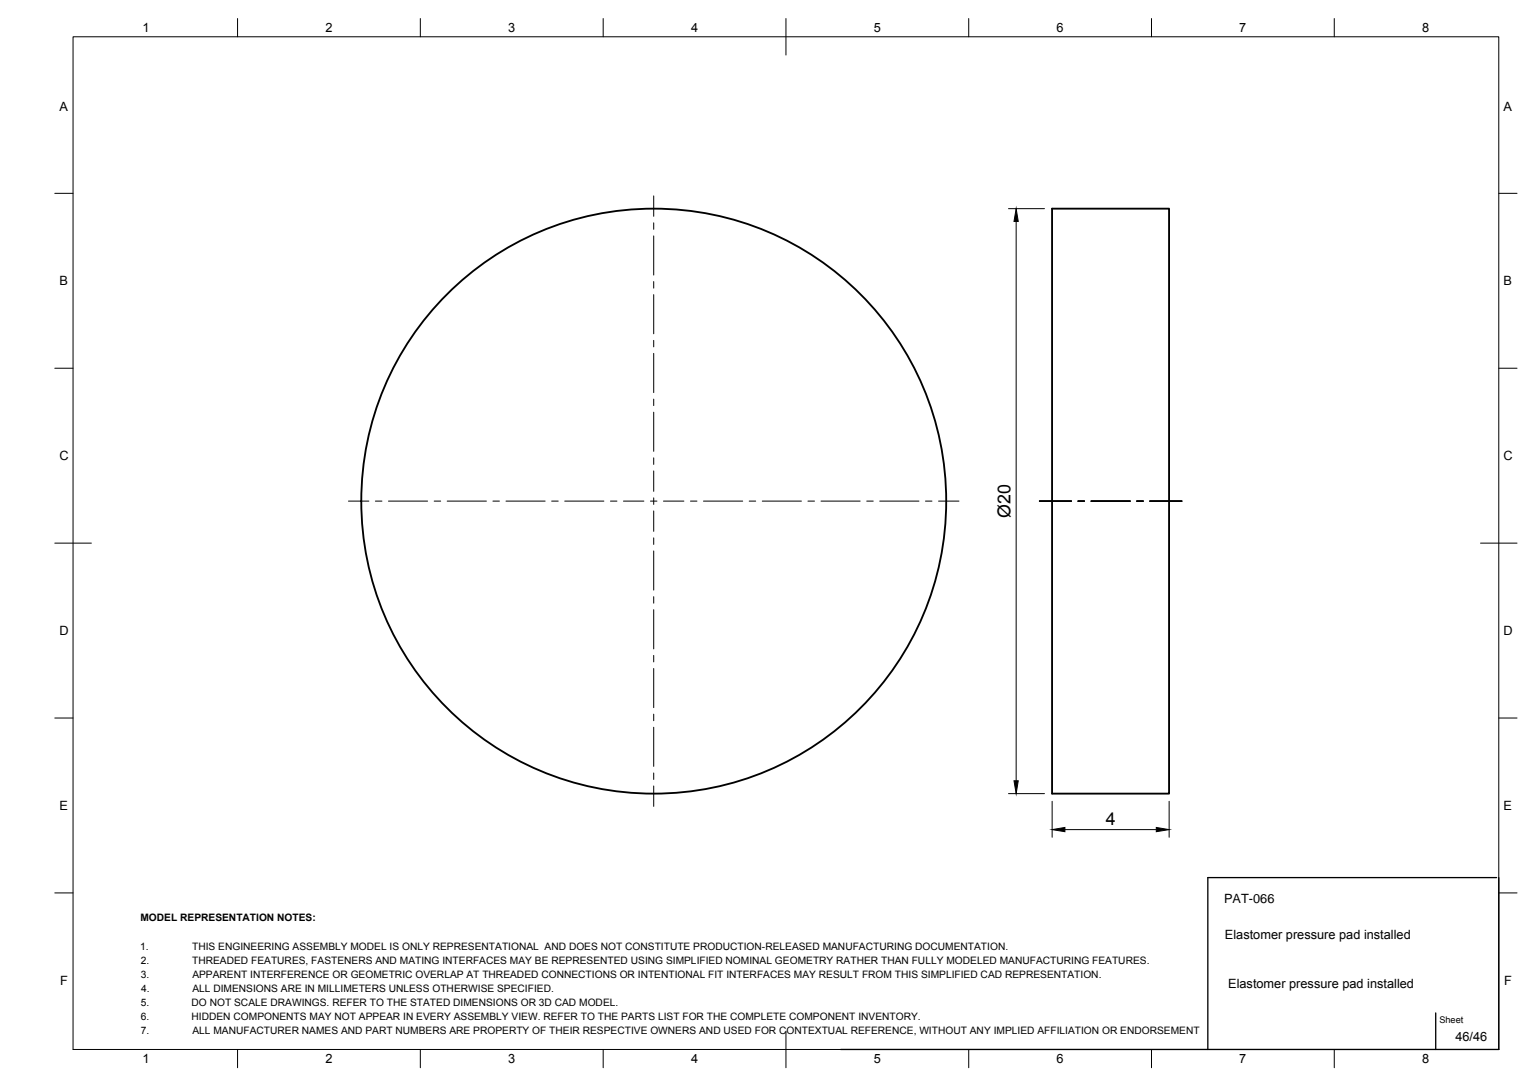
ISO-10303-21;
HEADER;
/* Generated by software containing ST-Developer
 * from STEP Tools, Inc. (www.steptools.com) 
 */

FILE_DESCRIPTION(
/* description */ ('Lever-operated bar clamp (toggle)'),
/* implementation_level */ '2;1');

FILE_NAME(
/* name */ 'Elastomer pressure pad installed.step',
/* time_stamp */ '2026-10-28T03:25:02-07:00',
/* author */ (''),
/* organization */ (''),
/* preprocessor_version */ 'ST-DEVELOPER v20.2',
/* originating_system */ 'Autodesk Translation Framework v15.17.0.0',
/* authorisation */ '');

FILE_SCHEMA (('AUTOMOTIVE_DESIGN { 1 0 10303 214 3 1 1 }'));
ENDSEC;

DATA;
#10=MECHANICAL_DESIGN_GEOMETRIC_PRESENTATION_REPRESENTATION('',(#455),#12413);
#370=SHAPE_REPRESENTATION_RELATIONSHIP('SRR','None',#12614,#408);
#408=ADVANCED_BREP_SHAPE_REPRESENTATION('',(#498),#12411);
#455=STYLED_ITEM('',(#12883),#498);
#498=MANIFOLD_SOLID_BREP('Body1',#6618);
#877=PLANE('',#7867);
#878=PLANE('',#7868);
#1279=FACE_OUTER_BOUND('',#1835,.T.);
#1280=FACE_OUTER_BOUND('',#1836,.T.);
#1281=FACE_OUTER_BOUND('',#1837,.T.);
#1835=EDGE_LOOP('',(#5977,#5978,#5979,#5980));
#1836=EDGE_LOOP('',(#5981));
#1837=EDGE_LOOP('',(#5982));
#2270=LINE('',#12256,#2711);
#2711=VECTOR('',#9967,1.);
#3068=CIRCLE('',#7865,1.);
#3069=CIRCLE('',#7866,1.);
#3597=VERTEX_POINT('',#12253);
#3598=VERTEX_POINT('',#12255);
#4393=EDGE_CURVE('',#3597,#3597,#3068,.T.);
#4394=EDGE_CURVE('',#3597,#3598,#2270,.T.);
#4395=EDGE_CURVE('',#3598,#3598,#3069,.T.);
#5977=ORIENTED_EDGE('',*,*,#4393,.F.);
#5978=ORIENTED_EDGE('',*,*,#4394,.T.);
#5979=ORIENTED_EDGE('',*,*,#4395,.T.);
#5980=ORIENTED_EDGE('',*,*,#4394,.F.);
#5981=ORIENTED_EDGE('',*,*,#4393,.T.);
#5982=ORIENTED_EDGE('',*,*,#4395,.F.);
#6161=CYLINDRICAL_SURFACE('',#7864,1.);
#6554=ADVANCED_FACE('',(#1279),#6161,.T.);
#6555=ADVANCED_FACE('',(#1280),#877,.T.);
#6556=ADVANCED_FACE('',(#1281),#878,.F.);
#6618=CLOSED_SHELL('',(#6554,#6555,#6556));
#7863=AXIS2_PLACEMENT_3D('',#12251,#9961,#9962);
#7864=AXIS2_PLACEMENT_3D('',#12252,#9963,#9964);
#7865=AXIS2_PLACEMENT_3D('',#12254,#9965,#9966);
#7866=AXIS2_PLACEMENT_3D('',#12257,#9968,#9969);
#7867=AXIS2_PLACEMENT_3D('',#12258,#9970,#9971);
#7868=AXIS2_PLACEMENT_3D('',#12259,#9972,#9973);
#9961=DIRECTION('axis',(0.,0.,1.));
#9962=DIRECTION('refdir',(1.,0.,0.));
#9963=DIRECTION('center_axis',(0.,0.,1.));
#9964=DIRECTION('ref_axis',(1.,0.,0.));
#9965=DIRECTION('center_axis',(0.,0.,1.));
#9966=DIRECTION('ref_axis',(1.,0.,0.));
#9967=DIRECTION('',(0.,0.,-1.));
#9968=DIRECTION('center_axis',(0.,0.,1.));
#9969=DIRECTION('ref_axis',(1.,0.,0.));
#9970=DIRECTION('center_axis',(0.,0.,1.));
#9971=DIRECTION('ref_axis',(1.,0.,0.));
#9972=DIRECTION('center_axis',(0.,0.,1.));
#9973=DIRECTION('ref_axis',(1.,0.,0.));
#12251=CARTESIAN_POINT('',(0.,0.,0.));
#12252=CARTESIAN_POINT('Origin',(0.,0.,3.));
#12253=CARTESIAN_POINT('',(-1.,-1.22464679914735E-16,3.4));
#12254=CARTESIAN_POINT('Origin',(0.,0.,3.4));
#12255=CARTESIAN_POINT('',(-1.,-1.22464679914735E-16,3.));
#12256=CARTESIAN_POINT('',(-1.,-1.22464679914735E-16,3.));
#12257=CARTESIAN_POINT('Origin',(0.,0.,3.));
#12258=CARTESIAN_POINT('Origin',(0.,0.,3.4));
#12259=CARTESIAN_POINT('Origin',(0.,0.,3.));
#12365=UNCERTAINTY_MEASURE_WITH_UNIT(LENGTH_MEASURE(0.001),#12414,
'DISTANCE_ACCURACY_VALUE',
'Maximum model space distance between geometric entities at asserted c
onnectivities');
#12367=UNCERTAINTY_MEASURE_WITH_UNIT(LENGTH_MEASURE(0.001),#12414,
'DISTANCE_ACCURACY_VALUE',
'Maximum model space distance between geometric entities at asserted c
onnectivities');
#12411=(
GEOMETRIC_REPRESENTATION_CONTEXT(3)
GLOBAL_UNCERTAINTY_ASSIGNED_CONTEXT((#12365))
GLOBAL_UNIT_ASSIGNED_CONTEXT((#12414,#12416,#12417))
REPRESENTATION_CONTEXT('','3D')
);
#12413=(
GEOMETRIC_REPRESENTATION_CONTEXT(3)
GLOBAL_UNCERTAINTY_ASSIGNED_CONTEXT((#12367))
GLOBAL_UNIT_ASSIGNED_CONTEXT((#12414,#12416,#12417))
REPRESENTATION_CONTEXT('','3D')
);
#12414=(
LENGTH_UNIT()
NAMED_UNIT(*)
SI_UNIT(.CENTI.,.METRE.)
);
#12416=(
NAMED_UNIT(*)
PLANE_ANGLE_UNIT()
SI_UNIT($,.RADIAN.)
);
#12417=(
NAMED_UNIT(*)
SI_UNIT($,.STERADIAN.)
SOLID_ANGLE_UNIT()
);
#12461=SHAPE_DEFINITION_REPRESENTATION(#12561,#12614);
#12561=PRODUCT_DEFINITION_SHAPE('',$,#12660);
#12614=SHAPE_REPRESENTATION('',(#7863),#12411);
#12616=PRODUCT_DEFINITION_CONTEXT('part definition',#12753,'design');
#12660=PRODUCT_DEFINITION('Elastomer pressure pad installed',
'Elastomer pressure pad installed',#12705,#12616);
#12705=PRODUCT_DEFINITION_FORMATION('',$,#12798);
#12753=APPLICATION_CONTEXT(
'Core Data for Automotive Mechanical Design Process');
#12754=PRODUCT_CONTEXT('part definition',#12753,'mechanical');
#12798=PRODUCT('Elastomer pressure pad installed',
'Elastomer pressure pad installed','Elastomer pressure pad installed',(#12754));
#12877=COLOUR_RGB('Off White',0.89,0.88,0.83);
#12878=FILL_AREA_STYLE_COLOUR('',#12877);
#12879=FILL_AREA_STYLE('',(#12878));
#12880=SURFACE_STYLE_FILL_AREA(#12879);
#12881=SURFACE_SIDE_STYLE('',(#12880));
#12882=SURFACE_STYLE_USAGE(.BOTH.,#12881);
#12883=PRESENTATION_STYLE_ASSIGNMENT((#12882));
ENDSEC;
END-ISO-10303-21;
